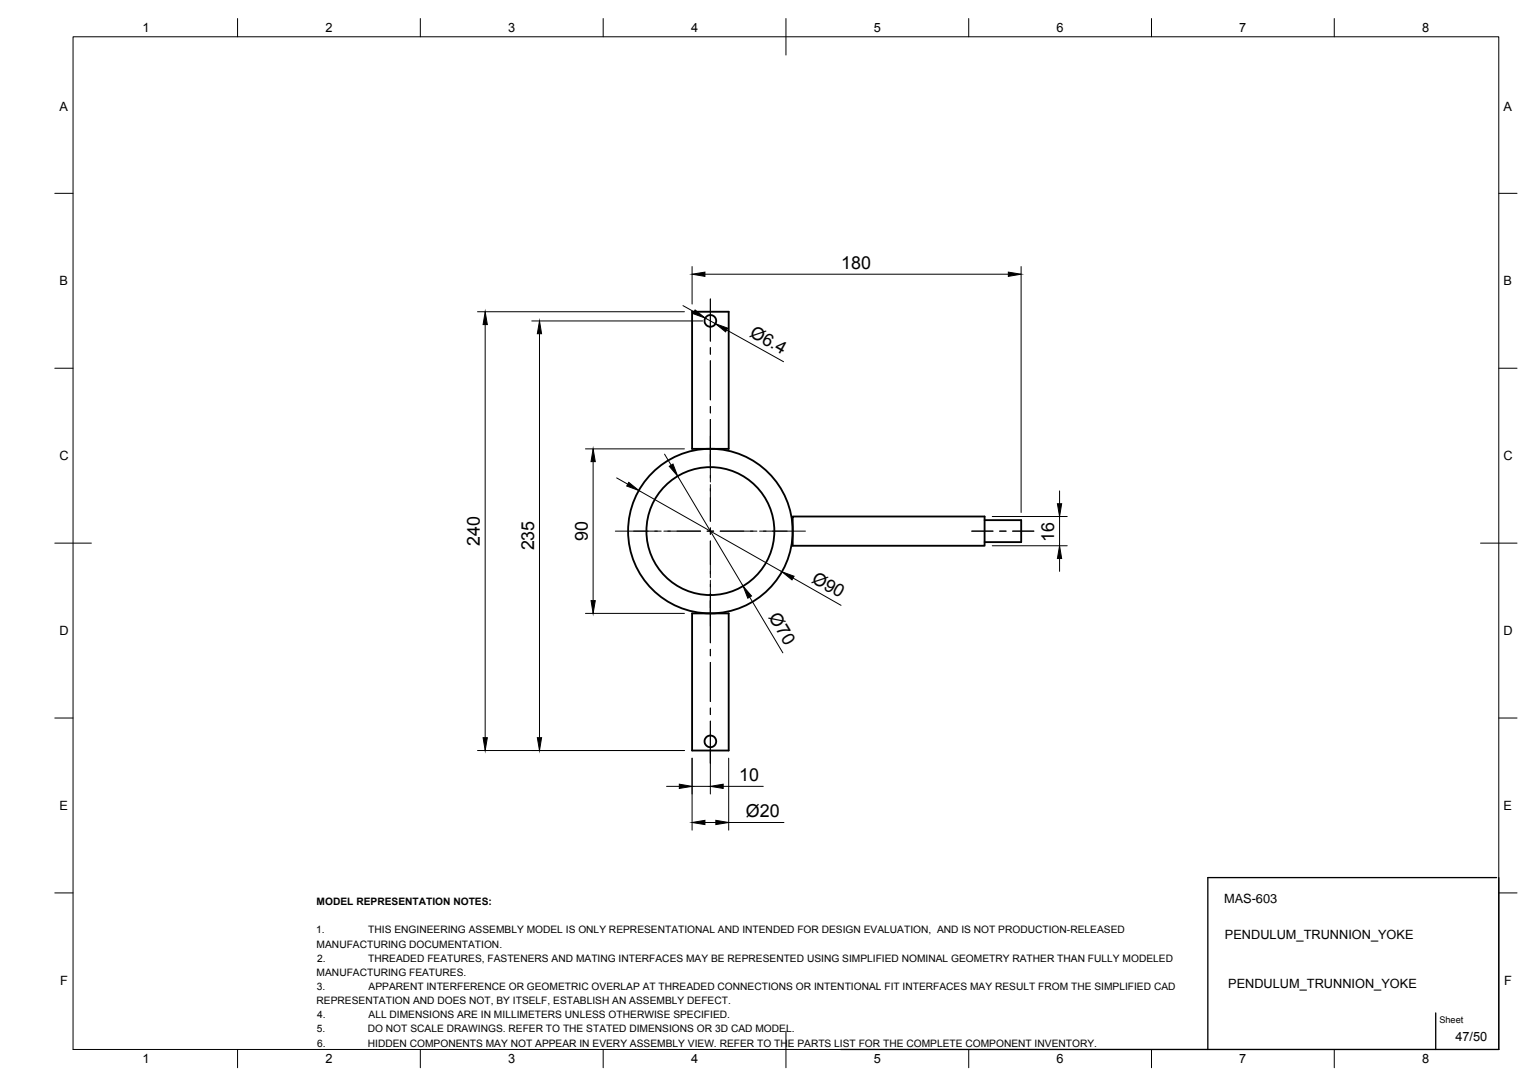
ISO-10303-21;
HEADER;
FILE_DESCRIPTION((''),'2;1');
FILE_NAME('PENDULUM_TRUNNION_YOKE.step','2026-10-01T22:06:14-07:00',(''),(''),'','','');
FILE_SCHEMA (('AUTOMOTIVE_DESIGN { 1 0 10303 214 3 1 1 }'));
ENDSEC;
DATA;
#10=MECHANICAL_DESIGN_GEOMETRIC_PRESENTATION_REPRESENTATION('',(#1022,#1023,#1024,#1025),#50440);
#38=B_SPLINE_CURVE_WITH_KNOTS('',3,(#49556,#49557,#49558,#49559,#49560,
#49561,#49562,#49563,#49564,#49565,#49566,#49567,#49568,#49569,#49570,#49571,
#49572,#49573,#49574),.UNSPECIFIED.,.F.,.F.,(4,2,2,2,3,2,2,2,4),(1.45762049263555,
1.57906514727215,1.70050980190876,1.82200189604475,1.94349399018073,2.06498608431671,
2.18647817845269,2.3079228330893,2.42936748772591),.UNSPECIFIED.) ;
#39=B_SPLINE_CURVE_WITH_KNOTS('',3,(#49577,#49578,#49579,#49580,#49581,
#49582,#49583,#49584,#49585,#49586,#49587,#49588,#49589,#49590,#49591,#49592,
#49593,#49594),.UNSPECIFIED.,.F.,.F.,(4,2,2,2,2,2,2,2,4),(0.485873497545182,
0.60731815218179,0.728762806818399,0.850254900954381,0.971746995090364,
1.09323908922635,1.21473118336233,1.33617583799894,1.45762049263555),
 .UNSPECIFIED.) ;
#40=B_SPLINE_CURVE_WITH_KNOTS('',3,(#49597,#49598,#49599,#49600,#49601,
#49602,#49603,#49604,#49605,#49606,#49607,#49608,#49609,#49610,#49611,#49612,
#49613,#49614),.UNSPECIFIED.,.F.,.F.,(4,2,2,2,2,2,2,2,4),(0.485873497545182,
0.607318152181791,0.728762806818399,0.850254900954382,0.971746995090364,
1.09323908922635,1.21473118336233,1.33617583799894,1.45762049263555),
 .UNSPECIFIED.) ;
#41=B_SPLINE_CURVE_WITH_KNOTS('',3,(#49615,#49616,#49617,#49618,#49619,
#49620,#49621,#49622,#49623,#49624,#49625,#49626,#49627,#49628,#49629,#49630,
#49631,#49632,#49633),.UNSPECIFIED.,.F.,.F.,(4,2,2,2,3,2,2,2,4),(1.45762049263555,
1.57906514727215,1.70050980190876,1.82200189604475,1.94349399018073,2.06498608431671,
2.18647817845269,2.3079228330893,2.42936748772591),.UNSPECIFIED.) ;
#42=B_SPLINE_CURVE_WITH_KNOTS('',3,(#49640,#49641,#49642,#49643,#49644,
#49645,#49646,#49647,#49648,#49649,#49650,#49651,#49652,#49653,#49654,#49655,
#49656,#49657),.UNSPECIFIED.,.F.,.F.,(4,2,2,2,2,2,2,2,4),(0.485873497545182,
0.607318152181791,0.728762806818399,0.850254900954382,0.971746995090364,
1.09323908922635,1.21473118336233,1.33617583799894,1.45762049263555),
 .UNSPECIFIED.) ;
#43=B_SPLINE_CURVE_WITH_KNOTS('',3,(#49658,#49659,#49660,#49661,#49662,
#49663,#49664,#49665,#49666,#49667,#49668,#49669,#49670,#49671,#49672,#49673,
#49674,#49675,#49676),.UNSPECIFIED.,.F.,.F.,(4,2,2,2,3,2,2,2,4),(1.45762049263555,
1.57906514727215,1.70050980190876,1.82200189604475,1.94349399018073,2.06498608431671,
2.18647817845269,2.3079228330893,2.42936748772591),.UNSPECIFIED.) ;
#44=B_SPLINE_CURVE_WITH_KNOTS('',3,(#49680,#49681,#49682,#49683,#49684,
#49685,#49686,#49687,#49688,#49689,#49690,#49691,#49692,#49693,#49694,#49695,
#49696,#49697,#49698),.UNSPECIFIED.,.F.,.F.,(4,2,2,2,3,2,2,2,4),(1.45762049263555,
1.57906514727215,1.70050980190876,1.82200189604475,1.94349399018073,2.06498608431671,
2.18647817845269,2.3079228330893,2.42936748772591),.UNSPECIFIED.) ;
#45=B_SPLINE_CURVE_WITH_KNOTS('',3,(#49699,#49700,#49701,#49702,#49703,
#49704,#49705,#49706,#49707,#49708,#49709,#49710,#49711,#49712,#49713,#49714,
#49715,#49716),.UNSPECIFIED.,.F.,.F.,(4,2,2,2,2,2,2,2,4),(0.485873497545182,
0.60731815218179,0.728762806818399,0.850254900954381,0.971746995090364,
1.09323908922635,1.21473118336233,1.33617583799894,1.45762049263555),
 .UNSPECIFIED.) ;
#925=SHAPE_REPRESENTATION_RELATIONSHIP('SRR','None',#50659,#970) ;
#970=ADVANCED_BREP_SHAPE_REPRESENTATION('',(#1075,#1076,#1077,#1078),#50428) ;
#1022=STYLED_ITEM('',(#50883),#1075) ;
#1023=STYLED_ITEM('',(#50883),#1076) ;
#1024=STYLED_ITEM('',(#50883),#1077) ;
#1025=STYLED_ITEM('',(#50883),#1078) ;
#1075=MANIFOLD_SOLID_BREP('PENDULUM_TRUNNION_YOKE',#28700) ;
#1076=MANIFOLD_SOLID_BREP('PENDULUM_TRUNNION_YOKE',#28701) ;
#1077=MANIFOLD_SOLID_BREP('PENDULUM_TRUNNION_YOKE',#28702) ;
#1078=MANIFOLD_SOLID_BREP('PENDULUM_TRUNNION_YOKE',#28703) ;
#1390=FACE_BOUND('',#5605,.T.) ;
#1391=FACE_BOUND('',#5612,.T.) ;
#1392=FACE_BOUND('',#5618,.T.) ;
#1393=FACE_BOUND('',#5622,.T.) ;
#1394=FACE_BOUND('',#5624,.T.) ;
#1395=FACE_BOUND('',#5626,.T.) ;
#2258=PLANE('',#32122) ;
#2259=PLANE('',#32123) ;
#2260=PLANE('',#32124) ;
#2261=PLANE('',#32125) ;
#2262=PLANE('',#32126) ;
#2263=PLANE('',#32127) ;
#2264=PLANE('',#32128) ;
#2265=PLANE('',#32129) ;
#2266=PLANE('',#32130) ;
#2267=PLANE('',#32132) ;
#2268=PLANE('',#32136) ;
#2269=PLANE('',#32139) ;
#2270=PLANE('',#32144) ;
#2271=PLANE('',#32145) ;
#2272=PLANE('',#32149) ;
#2273=PLANE('',#32152) ;
#3767=FACE_OUTER_BOUND('',#5599,.T.) ;
#3768=FACE_OUTER_BOUND('',#5600,.T.) ;
#3769=FACE_OUTER_BOUND('',#5601,.T.) ;
#3770=FACE_OUTER_BOUND('',#5602,.T.) ;
#3771=FACE_OUTER_BOUND('',#5603,.T.) ;
#3772=FACE_OUTER_BOUND('',#5604,.T.) ;
#3773=FACE_OUTER_BOUND('',#5606,.T.) ;
#3774=FACE_OUTER_BOUND('',#5607,.T.) ;
#3775=FACE_OUTER_BOUND('',#5608,.T.) ;
#3776=FACE_OUTER_BOUND('',#5609,.T.) ;
#3777=FACE_OUTER_BOUND('',#5610,.T.) ;
#3778=FACE_OUTER_BOUND('',#5611,.T.) ;
#3779=FACE_OUTER_BOUND('',#5613,.T.) ;
#3780=FACE_OUTER_BOUND('',#5614,.T.) ;
#3781=FACE_OUTER_BOUND('',#5615,.T.) ;
#3782=FACE_OUTER_BOUND('',#5616,.T.) ;
#3783=FACE_OUTER_BOUND('',#5617,.T.) ;
#3784=FACE_OUTER_BOUND('',#5619,.T.) ;
#3785=FACE_OUTER_BOUND('',#5620,.T.) ;
#3786=FACE_OUTER_BOUND('',#5621,.T.) ;
#3787=FACE_OUTER_BOUND('',#5623,.T.) ;
#3788=FACE_OUTER_BOUND('',#5625,.T.) ;
#3789=FACE_OUTER_BOUND('',#5627,.T.) ;
#3790=FACE_OUTER_BOUND('',#5628,.T.) ;
#5599=EDGE_LOOP('',(#26079,#26080,#26081,#26082)) ;
#5600=EDGE_LOOP('',(#26083)) ;
#5601=EDGE_LOOP('',(#26084,#26085,#26086,#26087)) ;
#5602=EDGE_LOOP('',(#26088,#26089,#26090,#26091,#26092)) ;
#5603=EDGE_LOOP('',(#26093,#26094,#26095,#26096,#26097)) ;
#5604=EDGE_LOOP('',(#26098,#26099,#26100,#26101)) ;
#5605=EDGE_LOOP('',(#26102)) ;
#5606=EDGE_LOOP('',(#26103,#26104,#26105,#26106)) ;
#5607=EDGE_LOOP('',(#26107,#26108,#26109,#26110)) ;
#5608=EDGE_LOOP('',(#26111,#26112,#26113,#26114)) ;
#5609=EDGE_LOOP('',(#26115)) ;
#5610=EDGE_LOOP('',(#26116,#26117)) ;
#5611=EDGE_LOOP('',(#26118,#26119,#26120,#26121,#26122,#26123,#26124,#26125,
#26126)) ;
#5612=EDGE_LOOP('',(#26127,#26128)) ;
#5613=EDGE_LOOP('',(#26129,#26130)) ;
#5614=EDGE_LOOP('',(#26131,#26132,#26133,#26134,#26135,#26136)) ;
#5615=EDGE_LOOP('',(#26137,#26138,#26139,#26140,#26141,#26142)) ;
#5616=EDGE_LOOP('',(#26143,#26144)) ;
#5617=EDGE_LOOP('',(#26145,#26146,#26147,#26148,#26149,#26150,#26151,#26152,
#26153)) ;
#5618=EDGE_LOOP('',(#26154,#26155)) ;
#5619=EDGE_LOOP('',(#26156)) ;
#5620=EDGE_LOOP('',(#26157,#26158)) ;
#5621=EDGE_LOOP('',(#26159,#26160,#26161,#26162,#26163,#26164,#26165,#26166)) ;
#5622=EDGE_LOOP('',(#26167,#26168)) ;
#5623=EDGE_LOOP('',(#26169,#26170)) ;
#5624=EDGE_LOOP('',(#26171)) ;
#5625=EDGE_LOOP('',(#26172,#26173)) ;
#5626=EDGE_LOOP('',(#26174)) ;
#5627=EDGE_LOOP('',(#26175,#26176,#26177,#26178,#26179,#26180,#26181,#26182)) ;
#5628=EDGE_LOOP('',(#26183,#26184,#26185,#26186)) ;
#8043=LINE('',#49509,#10515) ;
#8044=LINE('',#49515,#10516) ;
#8045=LINE('',#49517,#10517) ;
#8046=LINE('',#49519,#10518) ;
#8047=LINE('',#49520,#10519) ;
#8048=LINE('',#49524,#10520) ;
#8049=LINE('',#49525,#10521) ;
#8050=LINE('',#49527,#10522) ;
#8051=LINE('',#49528,#10523) ;
#8052=LINE('',#49532,#10524) ;
#8053=LINE('',#49534,#10525) ;
#8054=LINE('',#49535,#10526) ;
#8055=LINE('',#49536,#10527) ;
#8056=LINE('',#49538,#10528) ;
#8057=LINE('',#49539,#10529) ;
#8058=LINE('',#49542,#10530) ;
#8059=LINE('',#49550,#10531) ;
#8060=LINE('',#49554,#10532) ;
#8061=LINE('',#49575,#10533) ;
#8062=LINE('',#49636,#10534) ;
#8063=LINE('',#49678,#10535) ;
#8064=LINE('',#49720,#10536) ;
#8065=LINE('',#49724,#10537) ;
#8066=LINE('',#49726,#10538) ;
#8067=LINE('',#49733,#10539) ;
#8068=LINE('',#49735,#10540) ;
#8069=LINE('',#49737,#10541) ;
#8070=LINE('',#49741,#10542) ;
#8071=LINE('',#49743,#10543) ;
#8072=LINE('',#49745,#10544) ;
#8073=LINE('',#49749,#10545) ;
#8074=LINE('',#49760,#10546) ;
#10515=VECTOR('',#40510,0.6) ;
#10516=VECTOR('',#40517,1.) ;
#10517=VECTOR('',#40518,1.) ;
#10518=VECTOR('',#40519,1.) ;
#10519=VECTOR('',#40520,1.) ;
#10520=VECTOR('',#40523,1.) ;
#10521=VECTOR('',#40524,1.) ;
#10522=VECTOR('',#40525,1.) ;
#10523=VECTOR('',#40526,1.) ;
#10524=VECTOR('',#40529,1.) ;
#10525=VECTOR('',#40530,1.) ;
#10526=VECTOR('',#40531,1.) ;
#10527=VECTOR('',#40532,1.) ;
#10528=VECTOR('',#40535,1.) ;
#10529=VECTOR('',#40536,1.) ;
#10530=VECTOR('',#40541,1.) ;
#10531=VECTOR('',#40550,1.) ;
#10532=VECTOR('',#40555,1.) ;
#10533=VECTOR('',#40556,1.) ;
#10534=VECTOR('',#40563,0.32) ;
#10535=VECTOR('',#40566,0.32) ;
#10536=VECTOR('',#40569,1.) ;
#10537=VECTOR('',#40576,1.) ;
#10538=VECTOR('',#40577,1.) ;
#10539=VECTOR('',#40586,4.5) ;
#10540=VECTOR('',#40587,1.) ;
#10541=VECTOR('',#40588,4.5) ;
#10542=VECTOR('',#40591,4.5) ;
#10543=VECTOR('',#40592,1.) ;
#10544=VECTOR('',#40593,4.5) ;
#10545=VECTOR('',#40596,1.) ;
#10546=VECTOR('',#40613,3.5) ;
#11777=CIRCLE('',#32120,0.6) ;
#11778=CIRCLE('',#32121,0.6) ;
#11779=CIRCLE('',#32131,1.) ;
#11780=CIRCLE('',#32133,1.) ;
#11781=CIRCLE('',#32135,1.) ;
#11782=CIRCLE('',#32140,1.) ;
#11783=CIRCLE('',#32142,1.) ;
#11784=CIRCLE('',#32143,1.) ;
#11785=CIRCLE('',#32147,4.5) ;
#11786=CIRCLE('',#32148,4.5) ;
#11787=CIRCLE('',#32150,4.5) ;
#11788=CIRCLE('',#32151,3.5) ;
#11789=CIRCLE('',#32153,4.5) ;
#11790=CIRCLE('',#32154,3.5) ;
#14370=VERTEX_POINT('',#49506) ;
#14371=VERTEX_POINT('',#49508) ;
#14372=VERTEX_POINT('',#49513) ;
#14373=VERTEX_POINT('',#49514) ;
#14374=VERTEX_POINT('',#49516) ;
#14375=VERTEX_POINT('',#49518) ;
#14376=VERTEX_POINT('',#49522) ;
#14377=VERTEX_POINT('',#49523) ;
#14378=VERTEX_POINT('',#49526) ;
#14379=VERTEX_POINT('',#49530) ;
#14380=VERTEX_POINT('',#49531) ;
#14381=VERTEX_POINT('',#49533) ;
#14382=VERTEX_POINT('',#49545) ;
#14383=VERTEX_POINT('',#49548) ;
#14384=VERTEX_POINT('',#49549) ;
#14385=VERTEX_POINT('',#49553) ;
#14386=VERTEX_POINT('',#49555) ;
#14387=VERTEX_POINT('',#49595) ;
#14388=VERTEX_POINT('',#49596) ;
#14389=VERTEX_POINT('',#49638) ;
#14390=VERTEX_POINT('',#49639) ;
#14391=VERTEX_POINT('',#49677) ;
#14392=VERTEX_POINT('',#49679) ;
#14393=VERTEX_POINT('',#49718) ;
#14394=VERTEX_POINT('',#49719) ;
#14395=VERTEX_POINT('',#49725) ;
#14396=VERTEX_POINT('',#49731) ;
#14397=VERTEX_POINT('',#49732) ;
#14398=VERTEX_POINT('',#49734) ;
#14399=VERTEX_POINT('',#49736) ;
#14400=VERTEX_POINT('',#49738) ;
#14401=VERTEX_POINT('',#49740) ;
#14402=VERTEX_POINT('',#49742) ;
#14403=VERTEX_POINT('',#49744) ;
#14404=VERTEX_POINT('',#49747) ;
#14405=VERTEX_POINT('',#49748) ;
#14406=VERTEX_POINT('',#49752) ;
#14407=VERTEX_POINT('',#49756) ;
#18305=EDGE_CURVE('',#14370,#14370,#11777,.T.) ;
#18306=EDGE_CURVE('',#14370,#14371,#8043,.T.) ;
#18307=EDGE_CURVE('',#14371,#14371,#11778,.T.) ;
#18308=EDGE_CURVE('',#14372,#14373,#8044,.T.) ;
#18309=EDGE_CURVE('',#14374,#14372,#8045,.T.) ;
#18310=EDGE_CURVE('',#14375,#14374,#8046,.T.) ;
#18311=EDGE_CURVE('',#14373,#14375,#8047,.T.) ;
#18312=EDGE_CURVE('',#14376,#14377,#8048,.T.) ;
#18313=EDGE_CURVE('',#14377,#14373,#8049,.T.) ;
#18314=EDGE_CURVE('',#14375,#14378,#8050,.T.) ;
#18315=EDGE_CURVE('',#14378,#14376,#8051,.T.) ;
#18316=EDGE_CURVE('',#14379,#14380,#8052,.T.) ;
#18317=EDGE_CURVE('',#14380,#14381,#8053,.T.) ;
#18318=EDGE_CURVE('',#14381,#14374,#8054,.T.) ;
#18319=EDGE_CURVE('',#14372,#14379,#8055,.T.) ;
#18320=EDGE_CURVE('',#14378,#14381,#8056,.T.) ;
#18321=EDGE_CURVE('',#14376,#14380,#8057,.T.) ;
#18322=EDGE_CURVE('',#14377,#14379,#8058,.T.) ;
#18323=EDGE_CURVE('',#14382,#14382,#11779,.T.) ;
#18324=EDGE_CURVE('',#14383,#14384,#8059,.T.) ;
#18325=EDGE_CURVE('',#14384,#14383,#11780,.T.) ;
#18326=EDGE_CURVE('',#14382,#14385,#8060,.T.) ;
#18327=EDGE_CURVE('',#14385,#14386,#38,.T.) ;
#18328=EDGE_CURVE('',#14386,#14384,#8061,.T.) ;
#18329=EDGE_CURVE('',#14383,#14384,#11781,.T.) ;
#18330=EDGE_CURVE('',#14386,#14385,#39,.T.) ;
#18331=EDGE_CURVE('',#14387,#14388,#40,.T.) ;
#18332=EDGE_CURVE('',#14388,#14387,#41,.T.) ;
#18333=EDGE_CURVE('',#14388,#14386,#8062,.T.) ;
#18334=EDGE_CURVE('',#14389,#14390,#42,.T.) ;
#18335=EDGE_CURVE('',#14390,#14389,#43,.T.) ;
#18336=EDGE_CURVE('',#14390,#14391,#8063,.T.) ;
#18337=EDGE_CURVE('',#14392,#14391,#44,.T.) ;
#18338=EDGE_CURVE('',#14391,#14392,#45,.T.) ;
#18339=EDGE_CURVE('',#14393,#14394,#8064,.T.) ;
#18340=EDGE_CURVE('',#14393,#14394,#11782,.T.) ;
#18341=EDGE_CURVE('',#14394,#14393,#11783,.T.) ;
#18342=EDGE_CURVE('',#14394,#14392,#8065,.T.) ;
#18343=EDGE_CURVE('',#14391,#14395,#8066,.T.) ;
#18344=EDGE_CURVE('',#14395,#14395,#11784,.T.) ;
#18345=EDGE_CURVE('',#14396,#14397,#8067,.T.) ;
#18346=EDGE_CURVE('',#14398,#14396,#8068,.T.) ;
#18347=EDGE_CURVE('',#14399,#14398,#8069,.T.) ;
#18348=EDGE_CURVE('',#14400,#14399,#11785,.T.) ;
#18349=EDGE_CURVE('',#14401,#14400,#8070,.T.) ;
#18350=EDGE_CURVE('',#14401,#14402,#8071,.T.) ;
#18351=EDGE_CURVE('',#14403,#14402,#8072,.T.) ;
#18352=EDGE_CURVE('',#14397,#14403,#11786,.T.) ;
#18353=EDGE_CURVE('',#14404,#14405,#8073,.T.) ;
#18354=EDGE_CURVE('',#14403,#14397,#11787,.T.) ;
#18355=EDGE_CURVE('',#14406,#14406,#11788,.T.) ;
#18356=EDGE_CURVE('',#14399,#14400,#11789,.T.) ;
#18357=EDGE_CURVE('',#14407,#14407,#11790,.T.) ;
#18358=EDGE_CURVE('',#14407,#14406,#8074,.T.) ;
#26079=ORIENTED_EDGE('',*,*,#18305,.F.) ;
#26080=ORIENTED_EDGE('',*,*,#18306,.T.) ;
#26081=ORIENTED_EDGE('',*,*,#18307,.F.) ;
#26082=ORIENTED_EDGE('',*,*,#18306,.F.) ;
#26083=ORIENTED_EDGE('',*,*,#18307,.T.) ;
#26084=ORIENTED_EDGE('',*,*,#18308,.F.) ;
#26085=ORIENTED_EDGE('',*,*,#18309,.F.) ;
#26086=ORIENTED_EDGE('',*,*,#18310,.F.) ;
#26087=ORIENTED_EDGE('',*,*,#18311,.F.) ;
#26088=ORIENTED_EDGE('',*,*,#18312,.T.) ;
#26089=ORIENTED_EDGE('',*,*,#18313,.T.) ;
#26090=ORIENTED_EDGE('',*,*,#18311,.T.) ;
#26091=ORIENTED_EDGE('',*,*,#18314,.T.) ;
#26092=ORIENTED_EDGE('',*,*,#18315,.T.) ;
#26093=ORIENTED_EDGE('',*,*,#18316,.T.) ;
#26094=ORIENTED_EDGE('',*,*,#18317,.T.) ;
#26095=ORIENTED_EDGE('',*,*,#18318,.T.) ;
#26096=ORIENTED_EDGE('',*,*,#18309,.T.) ;
#26097=ORIENTED_EDGE('',*,*,#18319,.T.) ;
#26098=ORIENTED_EDGE('',*,*,#18320,.T.) ;
#26099=ORIENTED_EDGE('',*,*,#18317,.F.) ;
#26100=ORIENTED_EDGE('',*,*,#18321,.F.) ;
#26101=ORIENTED_EDGE('',*,*,#18315,.F.) ;
#26102=ORIENTED_EDGE('',*,*,#18305,.T.) ;
#26103=ORIENTED_EDGE('',*,*,#18310,.T.) ;
#26104=ORIENTED_EDGE('',*,*,#18318,.F.) ;
#26105=ORIENTED_EDGE('',*,*,#18320,.F.) ;
#26106=ORIENTED_EDGE('',*,*,#18314,.F.) ;
#26107=ORIENTED_EDGE('',*,*,#18308,.T.) ;
#26108=ORIENTED_EDGE('',*,*,#18313,.F.) ;
#26109=ORIENTED_EDGE('',*,*,#18322,.T.) ;
#26110=ORIENTED_EDGE('',*,*,#18319,.F.) ;
#26111=ORIENTED_EDGE('',*,*,#18321,.T.) ;
#26112=ORIENTED_EDGE('',*,*,#18316,.F.) ;
#26113=ORIENTED_EDGE('',*,*,#18322,.F.) ;
#26114=ORIENTED_EDGE('',*,*,#18312,.F.) ;
#26115=ORIENTED_EDGE('',*,*,#18323,.T.) ;
#26116=ORIENTED_EDGE('',*,*,#18324,.T.) ;
#26117=ORIENTED_EDGE('',*,*,#18325,.T.) ;
#26118=ORIENTED_EDGE('',*,*,#18323,.F.) ;
#26119=ORIENTED_EDGE('',*,*,#18326,.T.) ;
#26120=ORIENTED_EDGE('',*,*,#18327,.T.) ;
#26121=ORIENTED_EDGE('',*,*,#18328,.T.) ;
#26122=ORIENTED_EDGE('',*,*,#18329,.F.) ;
#26123=ORIENTED_EDGE('',*,*,#18325,.F.) ;
#26124=ORIENTED_EDGE('',*,*,#18328,.F.) ;
#26125=ORIENTED_EDGE('',*,*,#18330,.T.) ;
#26126=ORIENTED_EDGE('',*,*,#18326,.F.) ;
#26127=ORIENTED_EDGE('',*,*,#18331,.T.) ;
#26128=ORIENTED_EDGE('',*,*,#18332,.T.) ;
#26129=ORIENTED_EDGE('',*,*,#18324,.F.) ;
#26130=ORIENTED_EDGE('',*,*,#18329,.T.) ;
#26131=ORIENTED_EDGE('',*,*,#18331,.F.) ;
#26132=ORIENTED_EDGE('',*,*,#18332,.F.) ;
#26133=ORIENTED_EDGE('',*,*,#18333,.T.) ;
#26134=ORIENTED_EDGE('',*,*,#18327,.F.) ;
#26135=ORIENTED_EDGE('',*,*,#18330,.F.) ;
#26136=ORIENTED_EDGE('',*,*,#18333,.F.) ;
#26137=ORIENTED_EDGE('',*,*,#18334,.F.) ;
#26138=ORIENTED_EDGE('',*,*,#18335,.F.) ;
#26139=ORIENTED_EDGE('',*,*,#18336,.T.) ;
#26140=ORIENTED_EDGE('',*,*,#18337,.F.) ;
#26141=ORIENTED_EDGE('',*,*,#18338,.F.) ;
#26142=ORIENTED_EDGE('',*,*,#18336,.F.) ;
#26143=ORIENTED_EDGE('',*,*,#18339,.F.) ;
#26144=ORIENTED_EDGE('',*,*,#18340,.T.) ;
#26145=ORIENTED_EDGE('',*,*,#18340,.F.) ;
#26146=ORIENTED_EDGE('',*,*,#18341,.F.) ;
#26147=ORIENTED_EDGE('',*,*,#18342,.T.) ;
#26148=ORIENTED_EDGE('',*,*,#18337,.T.) ;
#26149=ORIENTED_EDGE('',*,*,#18343,.T.) ;
#26150=ORIENTED_EDGE('',*,*,#18344,.F.) ;
#26151=ORIENTED_EDGE('',*,*,#18343,.F.) ;
#26152=ORIENTED_EDGE('',*,*,#18338,.T.) ;
#26153=ORIENTED_EDGE('',*,*,#18342,.F.) ;
#26154=ORIENTED_EDGE('',*,*,#18334,.T.) ;
#26155=ORIENTED_EDGE('',*,*,#18335,.T.) ;
#26156=ORIENTED_EDGE('',*,*,#18344,.T.) ;
#26157=ORIENTED_EDGE('',*,*,#18339,.T.) ;
#26158=ORIENTED_EDGE('',*,*,#18341,.T.) ;
#26159=ORIENTED_EDGE('',*,*,#18345,.F.) ;
#26160=ORIENTED_EDGE('',*,*,#18346,.F.) ;
#26161=ORIENTED_EDGE('',*,*,#18347,.F.) ;
#26162=ORIENTED_EDGE('',*,*,#18348,.F.) ;
#26163=ORIENTED_EDGE('',*,*,#18349,.F.) ;
#26164=ORIENTED_EDGE('',*,*,#18350,.T.) ;
#26165=ORIENTED_EDGE('',*,*,#18351,.F.) ;
#26166=ORIENTED_EDGE('',*,*,#18352,.F.) ;
#26167=ORIENTED_EDGE('',*,*,#18353,.T.) ;
#26168=ORIENTED_EDGE('',*,*,#18353,.F.) ;
#26169=ORIENTED_EDGE('',*,*,#18354,.T.) ;
#26170=ORIENTED_EDGE('',*,*,#18352,.T.) ;
#26171=ORIENTED_EDGE('',*,*,#18355,.T.) ;
#26172=ORIENTED_EDGE('',*,*,#18348,.T.) ;
#26173=ORIENTED_EDGE('',*,*,#18356,.T.) ;
#26174=ORIENTED_EDGE('',*,*,#18357,.T.) ;
#26175=ORIENTED_EDGE('',*,*,#18345,.T.) ;
#26176=ORIENTED_EDGE('',*,*,#18354,.F.) ;
#26177=ORIENTED_EDGE('',*,*,#18351,.T.) ;
#26178=ORIENTED_EDGE('',*,*,#18350,.F.) ;
#26179=ORIENTED_EDGE('',*,*,#18349,.T.) ;
#26180=ORIENTED_EDGE('',*,*,#18356,.F.) ;
#26181=ORIENTED_EDGE('',*,*,#18347,.T.) ;
#26182=ORIENTED_EDGE('',*,*,#18346,.T.) ;
#26183=ORIENTED_EDGE('',*,*,#18357,.F.) ;
#26184=ORIENTED_EDGE('',*,*,#18358,.T.) ;
#26185=ORIENTED_EDGE('',*,*,#18355,.F.) ;
#26186=ORIENTED_EDGE('',*,*,#18358,.F.) ;
#27041=CYLINDRICAL_SURFACE('',#32119,0.6) ;
#27042=CYLINDRICAL_SURFACE('',#32134,1.) ;
#27043=CYLINDRICAL_SURFACE('',#32137,0.32) ;
#27044=CYLINDRICAL_SURFACE('',#32138,0.32) ;
#27045=CYLINDRICAL_SURFACE('',#32141,1.) ;
#27046=CYLINDRICAL_SURFACE('',#32146,4.5) ;
#27047=CYLINDRICAL_SURFACE('',#32155,4.5) ;
#27048=CYLINDRICAL_SURFACE('',#32156,3.5) ;
#28502=ADVANCED_FACE('',(#3767),#27041,.T.) ;
#28503=ADVANCED_FACE('',(#3768),#2258,.T.) ;
#28504=ADVANCED_FACE('',(#3769),#2259,.F.) ;
#28505=ADVANCED_FACE('',(#3770),#2260,.T.) ;
#28506=ADVANCED_FACE('',(#3771),#2261,.F.) ;
#28507=ADVANCED_FACE('',(#3772,#1390),#2262,.F.) ;
#28508=ADVANCED_FACE('',(#3773),#2263,.F.) ;
#28509=ADVANCED_FACE('',(#3774),#2264,.F.) ;
#28510=ADVANCED_FACE('',(#3775),#2265,.F.) ;
#28511=ADVANCED_FACE('',(#3776),#2266,.T.) ;
#28512=ADVANCED_FACE('',(#3777),#2267,.T.) ;
#28513=ADVANCED_FACE('',(#3778,#1391),#27042,.T.) ;
#28514=ADVANCED_FACE('',(#3779),#2268,.T.) ;
#28515=ADVANCED_FACE('',(#3780),#27043,.F.) ;
#28516=ADVANCED_FACE('',(#3781),#27044,.F.) ;
#28517=ADVANCED_FACE('',(#3782),#2269,.T.) ;
#28518=ADVANCED_FACE('',(#3783,#1392),#27045,.T.) ;
#28519=ADVANCED_FACE('',(#3784),#2270,.T.) ;
#28520=ADVANCED_FACE('',(#3785),#2271,.T.) ;
#28521=ADVANCED_FACE('',(#3786,#1393),#27046,.T.) ;
#28522=ADVANCED_FACE('',(#3787,#1394),#2272,.T.) ;
#28523=ADVANCED_FACE('',(#3788,#1395),#2273,.T.) ;
#28524=ADVANCED_FACE('',(#3789),#27047,.T.) ;
#28525=ADVANCED_FACE('',(#3790),#27048,.F.) ;
#28700=CLOSED_SHELL('',(#28502,#28503,#28504,#28505,#28506,#28507,#28508,
#28509,#28510)) ;
#28701=CLOSED_SHELL('',(#28511,#28512,#28513,#28514,#28515)) ;
#28702=CLOSED_SHELL('',(#28516,#28517,#28518,#28519,#28520)) ;
#28703=CLOSED_SHELL('',(#28521,#28522,#28523,#28524,#28525)) ;
#32118=AXIS2_PLACEMENT_3D('',#49504,#40504,#40505) ;
#32119=AXIS2_PLACEMENT_3D('',#49505,#40506,#40507) ;
#32120=AXIS2_PLACEMENT_3D('',#49507,#40508,#40509) ;
#32121=AXIS2_PLACEMENT_3D('',#49510,#40511,#40512) ;
#32122=AXIS2_PLACEMENT_3D('',#49511,#40513,#40514) ;
#32123=AXIS2_PLACEMENT_3D('',#49512,#40515,#40516) ;
#32124=AXIS2_PLACEMENT_3D('',#49521,#40521,#40522) ;
#32125=AXIS2_PLACEMENT_3D('',#49529,#40527,#40528) ;
#32126=AXIS2_PLACEMENT_3D('',#49537,#40533,#40534) ;
#32127=AXIS2_PLACEMENT_3D('',#49540,#40537,#40538) ;
#32128=AXIS2_PLACEMENT_3D('',#49541,#40539,#40540) ;
#32129=AXIS2_PLACEMENT_3D('',#49543,#40542,#40543) ;
#32130=AXIS2_PLACEMENT_3D('',#49544,#40544,#40545) ;
#32131=AXIS2_PLACEMENT_3D('',#49546,#40546,#40547) ;
#32132=AXIS2_PLACEMENT_3D('',#49547,#40548,#40549) ;
#32133=AXIS2_PLACEMENT_3D('',#49551,#40551,#40552) ;
#32134=AXIS2_PLACEMENT_3D('',#49552,#40553,#40554) ;
#32135=AXIS2_PLACEMENT_3D('',#49576,#40557,#40558) ;
#32136=AXIS2_PLACEMENT_3D('',#49634,#40559,#40560) ;
#32137=AXIS2_PLACEMENT_3D('',#49635,#40561,#40562) ;
#32138=AXIS2_PLACEMENT_3D('',#49637,#40564,#40565) ;
#32139=AXIS2_PLACEMENT_3D('',#49717,#40567,#40568) ;
#32140=AXIS2_PLACEMENT_3D('',#49721,#40570,#40571) ;
#32141=AXIS2_PLACEMENT_3D('',#49722,#40572,#40573) ;
#32142=AXIS2_PLACEMENT_3D('',#49723,#40574,#40575) ;
#32143=AXIS2_PLACEMENT_3D('',#49727,#40578,#40579) ;
#32144=AXIS2_PLACEMENT_3D('',#49728,#40580,#40581) ;
#32145=AXIS2_PLACEMENT_3D('',#49729,#40582,#40583) ;
#32146=AXIS2_PLACEMENT_3D('',#49730,#40584,#40585) ;
#32147=AXIS2_PLACEMENT_3D('',#49739,#40589,#40590) ;
#32148=AXIS2_PLACEMENT_3D('',#49746,#40594,#40595) ;
#32149=AXIS2_PLACEMENT_3D('',#49750,#40597,#40598) ;
#32150=AXIS2_PLACEMENT_3D('',#49751,#40599,#40600) ;
#32151=AXIS2_PLACEMENT_3D('',#49753,#40601,#40602) ;
#32152=AXIS2_PLACEMENT_3D('',#49754,#40603,#40604) ;
#32153=AXIS2_PLACEMENT_3D('',#49755,#40605,#40606) ;
#32154=AXIS2_PLACEMENT_3D('',#49757,#40607,#40608) ;
#32155=AXIS2_PLACEMENT_3D('',#49758,#40609,#40610) ;
#32156=AXIS2_PLACEMENT_3D('',#49759,#40611,#40612) ;
#40504=DIRECTION('axis',(0.,0.,1.)) ;
#40505=DIRECTION('refdir',(1.,0.,0.)) ;
#40506=DIRECTION('center_axis',(0.,1.,0.)) ;
#40507=DIRECTION('ref_axis',(1.,0.,0.)) ;
#40508=DIRECTION('center_axis',(0.,1.,0.)) ;
#40509=DIRECTION('ref_axis',(1.,0.,0.)) ;
#40510=DIRECTION('',(0.,-1.,0.)) ;
#40511=DIRECTION('center_axis',(0.,-1.,0.)) ;
#40512=DIRECTION('ref_axis',(1.,0.,0.)) ;
#40513=DIRECTION('center_axis',(0.,-1.,0.)) ;
#40514=DIRECTION('ref_axis',(-1.,0.,0.)) ;
#40515=DIRECTION('center_axis',(0.,-1.,0.)) ;
#40516=DIRECTION('ref_axis',(0.,0.,-1.)) ;
#40517=DIRECTION('',(0.,0.,1.)) ;
#40518=DIRECTION('',(1.,0.,0.)) ;
#40519=DIRECTION('',(0.,0.,-1.)) ;
#40520=DIRECTION('',(-1.,0.,0.)) ;
#40521=DIRECTION('center_axis',(0.,0.,1.)) ;
#40522=DIRECTION('ref_axis',(1.,0.,0.)) ;
#40523=DIRECTION('',(0.,1.,0.)) ;
#40524=DIRECTION('',(-1.,0.,0.)) ;
#40525=DIRECTION('',(0.,-1.,0.)) ;
#40526=DIRECTION('',(1.,0.,0.)) ;
#40527=DIRECTION('center_axis',(0.,0.,1.)) ;
#40528=DIRECTION('ref_axis',(1.,0.,0.)) ;
#40529=DIRECTION('',(0.,-1.,0.)) ;
#40530=DIRECTION('',(-1.,0.,0.)) ;
#40531=DIRECTION('',(0.,1.,0.)) ;
#40532=DIRECTION('',(1.,0.,0.)) ;
#40533=DIRECTION('center_axis',(0.,1.,0.)) ;
#40534=DIRECTION('ref_axis',(0.,0.,1.)) ;
#40535=DIRECTION('',(0.,0.,-1.)) ;
#40536=DIRECTION('',(0.,0.,-1.)) ;
#40537=DIRECTION('center_axis',(1.,0.,0.)) ;
#40538=DIRECTION('ref_axis',(0.,0.,-1.)) ;
#40539=DIRECTION('center_axis',(0.,-1.,0.)) ;
#40540=DIRECTION('ref_axis',(0.,0.,-1.)) ;
#40541=DIRECTION('',(0.,0.,-1.)) ;
#40542=DIRECTION('center_axis',(-1.,0.,0.)) ;
#40543=DIRECTION('ref_axis',(0.,0.,1.)) ;
#40544=DIRECTION('center_axis',(1.,0.,0.)) ;
#40545=DIRECTION('ref_axis',(0.,0.,-1.)) ;
#40546=DIRECTION('center_axis',(1.,0.,0.)) ;
#40547=DIRECTION('ref_axis',(0.,0.,-1.)) ;
#40548=DIRECTION('center_axis',(-1.,0.,0.)) ;
#40549=DIRECTION('ref_axis',(0.,0.,1.)) ;
#40550=DIRECTION('',(0.,0.,1.)) ;
#40551=DIRECTION('center_axis',(-1.,0.,0.)) ;
#40552=DIRECTION('ref_axis',(0.,0.,-1.)) ;
#40553=DIRECTION('center_axis',(1.,0.,0.)) ;
#40554=DIRECTION('ref_axis',(0.,0.,-1.)) ;
#40555=DIRECTION('',(-1.,0.,0.)) ;
#40556=DIRECTION('',(-1.,0.,0.)) ;
#40557=DIRECTION('center_axis',(-1.,0.,0.)) ;
#40558=DIRECTION('ref_axis',(0.,0.,-1.)) ;
#40559=DIRECTION('center_axis',(-1.,0.,0.)) ;
#40560=DIRECTION('ref_axis',(0.,0.,1.)) ;
#40561=DIRECTION('center_axis',(0.,0.,1.)) ;
#40562=DIRECTION('ref_axis',(1.,0.,0.)) ;
#40563=DIRECTION('',(0.,0.,1.)) ;
#40564=DIRECTION('center_axis',(0.,0.,1.)) ;
#40565=DIRECTION('ref_axis',(1.,0.,0.)) ;
#40566=DIRECTION('',(0.,0.,1.)) ;
#40567=DIRECTION('center_axis',(1.,0.,0.)) ;
#40568=DIRECTION('ref_axis',(0.,0.,-1.)) ;
#40569=DIRECTION('',(0.,0.,1.)) ;
#40570=DIRECTION('center_axis',(1.,0.,0.)) ;
#40571=DIRECTION('ref_axis',(0.,0.,-1.)) ;
#40572=DIRECTION('center_axis',(1.,0.,0.)) ;
#40573=DIRECTION('ref_axis',(0.,0.,-1.)) ;
#40574=DIRECTION('center_axis',(1.,0.,0.)) ;
#40575=DIRECTION('ref_axis',(0.,0.,-1.)) ;
#40576=DIRECTION('',(-1.,0.,0.)) ;
#40577=DIRECTION('',(-1.,0.,0.)) ;
#40578=DIRECTION('center_axis',(-1.,0.,0.)) ;
#40579=DIRECTION('ref_axis',(0.,0.,-1.)) ;
#40580=DIRECTION('center_axis',(-1.,0.,0.)) ;
#40581=DIRECTION('ref_axis',(0.,0.,1.)) ;
#40582=DIRECTION('center_axis',(1.,0.,0.)) ;
#40583=DIRECTION('ref_axis',(0.,0.,-1.)) ;
#40584=DIRECTION('center_axis',(0.,0.,1.)) ;
#40585=DIRECTION('ref_axis',(6.12323399573677E-17,1.,0.)) ;
#40586=DIRECTION('',(0.,0.,1.)) ;
#40587=DIRECTION('',(0.,0.,1.)) ;
#40588=DIRECTION('',(0.,0.,1.)) ;
#40589=DIRECTION('center_axis',(0.,0.,-1.)) ;
#40590=DIRECTION('ref_axis',(1.,0.,0.)) ;
#40591=DIRECTION('',(0.,0.,-1.)) ;
#40592=DIRECTION('',(0.,0.,1.)) ;
#40593=DIRECTION('',(0.,0.,-1.)) ;
#40594=DIRECTION('center_axis',(0.,0.,1.)) ;
#40595=DIRECTION('ref_axis',(1.,0.,0.)) ;
#40596=DIRECTION('',(0.,0.,1.)) ;
#40597=DIRECTION('center_axis',(0.,0.,1.)) ;
#40598=DIRECTION('ref_axis',(1.,0.,0.)) ;
#40599=DIRECTION('center_axis',(0.,0.,1.)) ;
#40600=DIRECTION('ref_axis',(1.,0.,0.)) ;
#40601=DIRECTION('center_axis',(0.,0.,-1.)) ;
#40602=DIRECTION('ref_axis',(1.,0.,0.)) ;
#40603=DIRECTION('center_axis',(0.,0.,-1.)) ;
#40604=DIRECTION('ref_axis',(-1.,0.,0.)) ;
#40605=DIRECTION('center_axis',(0.,0.,-1.)) ;
#40606=DIRECTION('ref_axis',(1.,0.,0.)) ;
#40607=DIRECTION('center_axis',(0.,0.,1.)) ;
#40608=DIRECTION('ref_axis',(1.,0.,0.)) ;
#40609=DIRECTION('center_axis',(0.,0.,1.)) ;
#40610=DIRECTION('ref_axis',(6.12323399573677E-17,1.,0.)) ;
#40611=DIRECTION('center_axis',(0.,0.,1.)) ;
#40612=DIRECTION('ref_axis',(1.,0.,0.)) ;
#40613=DIRECTION('',(0.,0.,1.)) ;
#49504=CARTESIAN_POINT('',(0.,0.,0.)) ;
#49505=CARTESIAN_POINT('Origin',(0.,-16.,24.)) ;
#49506=CARTESIAN_POINT('',(-0.6,-15.,24.)) ;
#49507=CARTESIAN_POINT('Origin',(0.,-15.,24.)) ;
#49508=CARTESIAN_POINT('',(-0.6,-17.,24.)) ;
#49509=CARTESIAN_POINT('',(-0.6,-16.,24.)) ;
#49510=CARTESIAN_POINT('Origin',(0.,-17.,24.)) ;
#49511=CARTESIAN_POINT('Origin',(0.,-17.,24.)) ;
#49512=CARTESIAN_POINT('Origin',(0.,-4.5,24.)) ;
#49513=CARTESIAN_POINT('',(0.,-4.5,23.2)) ;
#49514=CARTESIAN_POINT('',(0.,-4.5,24.8)) ;
#49515=CARTESIAN_POINT('',(0.,-4.5,24.)) ;
#49516=CARTESIAN_POINT('',(-0.8,-4.5,23.2)) ;
#49517=CARTESIAN_POINT('',(0.,-4.5,23.2)) ;
#49518=CARTESIAN_POINT('',(-0.8,-4.5,24.8)) ;
#49519=CARTESIAN_POINT('',(-0.8,-4.5,24.)) ;
#49520=CARTESIAN_POINT('',(0.,-4.5,24.8)) ;
#49521=CARTESIAN_POINT('Origin',(0.,-9.75,24.8)) ;
#49522=CARTESIAN_POINT('',(0.8,-15.,24.8)) ;
#49523=CARTESIAN_POINT('',(0.8,-4.5,24.8)) ;
#49524=CARTESIAN_POINT('',(0.8,-9.75,24.8)) ;
#49525=CARTESIAN_POINT('',(0.,-4.5,24.8)) ;
#49526=CARTESIAN_POINT('',(-0.8,-15.,24.8)) ;
#49527=CARTESIAN_POINT('',(-0.8,-9.75,24.8)) ;
#49528=CARTESIAN_POINT('',(0.,-15.,24.8)) ;
#49529=CARTESIAN_POINT('Origin',(0.,-9.75,23.2)) ;
#49530=CARTESIAN_POINT('',(0.8,-4.5,23.2)) ;
#49531=CARTESIAN_POINT('',(0.8,-15.,23.2)) ;
#49532=CARTESIAN_POINT('',(0.8,-9.75,23.2)) ;
#49533=CARTESIAN_POINT('',(-0.8,-15.,23.2)) ;
#49534=CARTESIAN_POINT('',(0.,-15.,23.2)) ;
#49535=CARTESIAN_POINT('',(-0.8,-9.75,23.2)) ;
#49536=CARTESIAN_POINT('',(0.,-4.5,23.2)) ;
#49537=CARTESIAN_POINT('Origin',(0.,-15.,24.)) ;
#49538=CARTESIAN_POINT('',(-0.8,-15.,24.)) ;
#49539=CARTESIAN_POINT('',(0.8,-15.,24.)) ;
#49540=CARTESIAN_POINT('Origin',(-0.8,-9.75,24.)) ;
#49541=CARTESIAN_POINT('Origin',(0.,-4.5,24.)) ;
#49542=CARTESIAN_POINT('',(0.8,-4.5,24.)) ;
#49543=CARTESIAN_POINT('Origin',(0.8,-9.75,24.)) ;
#49544=CARTESIAN_POINT('Origin',(12.,0.,24.)) ;
#49545=CARTESIAN_POINT('',(12.,-1.22464679914735E-16,25.)) ;
#49546=CARTESIAN_POINT('Origin',(12.,0.,24.)) ;
#49547=CARTESIAN_POINT('Origin',(4.5,0.,24.)) ;
#49548=CARTESIAN_POINT('',(4.5,0.,23.)) ;
#49549=CARTESIAN_POINT('',(4.5,0.,25.)) ;
#49550=CARTESIAN_POINT('',(4.5,0.,24.)) ;
#49551=CARTESIAN_POINT('Origin',(4.5,0.,24.)) ;
#49552=CARTESIAN_POINT('Origin',(8.25,0.,24.)) ;
#49553=CARTESIAN_POINT('',(11.82,0.,25.)) ;
#49554=CARTESIAN_POINT('',(8.25,-1.22464679914735E-16,25.)) ;
#49555=CARTESIAN_POINT('',(11.18,0.,25.)) ;
#49556=CARTESIAN_POINT('Ctrl Pts',(11.82,0.,25.)) ;
#49557=CARTESIAN_POINT('Ctrl Pts',(11.82,-0.0404815515455362,25.)) ;
#49558=CARTESIAN_POINT('Ctrl Pts',(11.8118517942692,-0.0834711465257763,
24.9972999591064)) ;
#49559=CARTESIAN_POINT('Ctrl Pts',(11.7791044225004,-0.162233452253763,
24.9875499722835)) ;
#49560=CARTESIAN_POINT('Ctrl Pts',(11.7545204234507,-0.198027916508675,
24.9806252339521)) ;
#49561=CARTESIAN_POINT('Ctrl Pts',(11.6980168827738,-0.254531457185612,
24.9674995088223)) ;
#49562=CARTESIAN_POINT('Ctrl Pts',(11.6622268501742,-0.279106940985719,
24.9604129001751)) ;
#49563=CARTESIAN_POINT('Ctrl Pts',(11.583480842843,-0.311847989268857,24.9502865189927)) ;
#49564=CARTESIAN_POINT('Ctrl Pts',(11.540497364712,-0.32,24.9474175425862)) ;
#49565=CARTESIAN_POINT('Ctrl Pts',(11.5,-0.32,24.9474175425862)) ;
#49566=CARTESIAN_POINT('Ctrl Pts',(11.459502635288,-0.32,24.9474175425862)) ;
#49567=CARTESIAN_POINT('Ctrl Pts',(11.416519157157,-0.311847989268857,24.9502865189927)) ;
#49568=CARTESIAN_POINT('Ctrl Pts',(11.3377731498258,-0.279106940985719,
24.9604129001751)) ;
#49569=CARTESIAN_POINT('Ctrl Pts',(11.3019831172262,-0.254531457185612,
24.9674995088223)) ;
#49570=CARTESIAN_POINT('Ctrl Pts',(11.2454795765493,-0.198027916508675,
24.9806252339521)) ;
#49571=CARTESIAN_POINT('Ctrl Pts',(11.2208955774996,-0.162233452253763,
24.9875499722835)) ;
#49572=CARTESIAN_POINT('Ctrl Pts',(11.1881482057308,-0.0834711465257753,
24.9972999591064)) ;
#49573=CARTESIAN_POINT('Ctrl Pts',(11.18,-0.0404815515455361,25.)) ;
#49574=CARTESIAN_POINT('Ctrl Pts',(11.18,8.32667268468867E-17,25.)) ;
#49575=CARTESIAN_POINT('',(8.25,-1.22464679914735E-16,25.)) ;
#49576=CARTESIAN_POINT('Origin',(4.5,0.,24.)) ;
#49577=CARTESIAN_POINT('Ctrl Pts',(11.18,7.63278329429795E-17,25.)) ;
#49578=CARTESIAN_POINT('Ctrl Pts',(11.18,0.0404815515455362,25.)) ;
#49579=CARTESIAN_POINT('Ctrl Pts',(11.1881482057308,0.0834711465257764,
24.9972999591064)) ;
#49580=CARTESIAN_POINT('Ctrl Pts',(11.2208955774996,0.162233452253763,24.9875499722835)) ;
#49581=CARTESIAN_POINT('Ctrl Pts',(11.2454795765493,0.198027916508675,24.9806252339521)) ;
#49582=CARTESIAN_POINT('Ctrl Pts',(11.3019831172262,0.254531457185612,24.9674995088223)) ;
#49583=CARTESIAN_POINT('Ctrl Pts',(11.3377731498258,0.279106940985719,24.9604129001751)) ;
#49584=CARTESIAN_POINT('Ctrl Pts',(11.416519157157,0.311847989268857,24.9502865189927)) ;
#49585=CARTESIAN_POINT('Ctrl Pts',(11.459502635288,0.32,24.9474175425862)) ;
#49586=CARTESIAN_POINT('Ctrl Pts',(11.540497364712,0.32,24.9474175425862)) ;
#49587=CARTESIAN_POINT('Ctrl Pts',(11.583480842843,0.311847989268857,24.9502865189927)) ;
#49588=CARTESIAN_POINT('Ctrl Pts',(11.6622268501742,0.279106940985719,24.9604129001751)) ;
#49589=CARTESIAN_POINT('Ctrl Pts',(11.6980168827738,0.254531457185612,24.9674995088223)) ;
#49590=CARTESIAN_POINT('Ctrl Pts',(11.7545204234507,0.198027916508675,24.9806252339521)) ;
#49591=CARTESIAN_POINT('Ctrl Pts',(11.7791044225004,0.162233452253763,24.9875499722835)) ;
#49592=CARTESIAN_POINT('Ctrl Pts',(11.8118517942692,0.0834711465257763,
24.9972999591064)) ;
#49593=CARTESIAN_POINT('Ctrl Pts',(11.82,0.0404815515455362,25.)) ;
#49594=CARTESIAN_POINT('Ctrl Pts',(11.82,0.,25.)) ;
#49595=CARTESIAN_POINT('',(11.82,0.,23.)) ;
#49596=CARTESIAN_POINT('',(11.18,0.,23.)) ;
#49597=CARTESIAN_POINT('Ctrl Pts',(11.82,-6.93889390390723E-17,23.)) ;
#49598=CARTESIAN_POINT('Ctrl Pts',(11.82,0.0404815515455361,23.)) ;
#49599=CARTESIAN_POINT('Ctrl Pts',(11.8118517942692,0.0834711465257763,
23.0027000408936)) ;
#49600=CARTESIAN_POINT('Ctrl Pts',(11.7791044225004,0.162233452253763,23.0124500277165)) ;
#49601=CARTESIAN_POINT('Ctrl Pts',(11.7545204234507,0.198027916508675,23.0193747660479)) ;
#49602=CARTESIAN_POINT('Ctrl Pts',(11.6980168827738,0.254531457185612,23.0325004911777)) ;
#49603=CARTESIAN_POINT('Ctrl Pts',(11.6622268501742,0.279106940985719,23.0395870998249)) ;
#49604=CARTESIAN_POINT('Ctrl Pts',(11.583480842843,0.311847989268857,23.0497134810073)) ;
#49605=CARTESIAN_POINT('Ctrl Pts',(11.540497364712,0.32,23.0525824574138)) ;
#49606=CARTESIAN_POINT('Ctrl Pts',(11.459502635288,0.32,23.0525824574138)) ;
#49607=CARTESIAN_POINT('Ctrl Pts',(11.416519157157,0.311847989268857,23.0497134810073)) ;
#49608=CARTESIAN_POINT('Ctrl Pts',(11.3377731498258,0.279106940985719,23.0395870998249)) ;
#49609=CARTESIAN_POINT('Ctrl Pts',(11.3019831172262,0.254531457185612,23.0325004911777)) ;
#49610=CARTESIAN_POINT('Ctrl Pts',(11.2454795765493,0.198027916508675,23.0193747660479)) ;
#49611=CARTESIAN_POINT('Ctrl Pts',(11.2208955774996,0.162233452253763,23.0124500277165)) ;
#49612=CARTESIAN_POINT('Ctrl Pts',(11.1881482057308,0.0834711465257763,
23.0027000408936)) ;
#49613=CARTESIAN_POINT('Ctrl Pts',(11.18,0.0404815515455361,23.)) ;
#49614=CARTESIAN_POINT('Ctrl Pts',(11.18,0.,23.)) ;
#49615=CARTESIAN_POINT('Ctrl Pts',(11.18,1.80411241501588E-16,23.)) ;
#49616=CARTESIAN_POINT('Ctrl Pts',(11.18,-0.040481551545536,23.)) ;
#49617=CARTESIAN_POINT('Ctrl Pts',(11.1881482057308,-0.0834711465257763,
23.0027000408936)) ;
#49618=CARTESIAN_POINT('Ctrl Pts',(11.2208955774996,-0.162233452253763,
23.0124500277165)) ;
#49619=CARTESIAN_POINT('Ctrl Pts',(11.2454795765493,-0.198027916508675,
23.0193747660479)) ;
#49620=CARTESIAN_POINT('Ctrl Pts',(11.3019831172262,-0.254531457185612,
23.0325004911777)) ;
#49621=CARTESIAN_POINT('Ctrl Pts',(11.3377731498258,-0.279106940985719,
23.0395870998249)) ;
#49622=CARTESIAN_POINT('Ctrl Pts',(11.416519157157,-0.311847989268857,23.0497134810073)) ;
#49623=CARTESIAN_POINT('Ctrl Pts',(11.459502635288,-0.32,23.0525824574138)) ;
#49624=CARTESIAN_POINT('Ctrl Pts',(11.5,-0.32,23.0525824574138)) ;
#49625=CARTESIAN_POINT('Ctrl Pts',(11.540497364712,-0.32,23.0525824574138)) ;
#49626=CARTESIAN_POINT('Ctrl Pts',(11.583480842843,-0.311847989268857,23.0497134810073)) ;
#49627=CARTESIAN_POINT('Ctrl Pts',(11.6622268501742,-0.279106940985719,
23.0395870998249)) ;
#49628=CARTESIAN_POINT('Ctrl Pts',(11.6980168827738,-0.254531457185612,
23.0325004911777)) ;
#49629=CARTESIAN_POINT('Ctrl Pts',(11.7545204234507,-0.198027916508675,
23.0193747660479)) ;
#49630=CARTESIAN_POINT('Ctrl Pts',(11.7791044225004,-0.162233452253763,
23.0124500277165)) ;
#49631=CARTESIAN_POINT('Ctrl Pts',(11.8118517942692,-0.0834711465257763,
23.0027000408936)) ;
#49632=CARTESIAN_POINT('Ctrl Pts',(11.82,-0.0404815515455362,23.)) ;
#49633=CARTESIAN_POINT('Ctrl Pts',(11.82,-6.93889390390723E-18,23.)) ;
#49634=CARTESIAN_POINT('Origin',(4.5,0.,24.)) ;
#49635=CARTESIAN_POINT('Origin',(11.5,0.,24.)) ;
#49636=CARTESIAN_POINT('',(11.18,-3.91886975727153E-17,24.)) ;
#49637=CARTESIAN_POINT('Origin',(-11.5,0.,24.)) ;
#49638=CARTESIAN_POINT('',(-11.18,0.,23.)) ;
#49639=CARTESIAN_POINT('',(-11.82,0.,23.)) ;
#49640=CARTESIAN_POINT('Ctrl Pts',(-11.18,-6.24500451351651E-17,23.)) ;
#49641=CARTESIAN_POINT('Ctrl Pts',(-11.18,0.0404815515455361,23.)) ;
#49642=CARTESIAN_POINT('Ctrl Pts',(-11.1881482057308,0.0834711465257763,
23.0027000408936)) ;
#49643=CARTESIAN_POINT('Ctrl Pts',(-11.2208955774996,0.162233452253763,
23.0124500277165)) ;
#49644=CARTESIAN_POINT('Ctrl Pts',(-11.2454795765493,0.198027916508675,
23.0193747660479)) ;
#49645=CARTESIAN_POINT('Ctrl Pts',(-11.3019831172262,0.254531457185612,
23.0325004911777)) ;
#49646=CARTESIAN_POINT('Ctrl Pts',(-11.3377731498258,0.279106940985719,
23.0395870998249)) ;
#49647=CARTESIAN_POINT('Ctrl Pts',(-11.416519157157,0.311847989268857,23.0497134810073)) ;
#49648=CARTESIAN_POINT('Ctrl Pts',(-11.459502635288,0.32,23.0525824574138)) ;
#49649=CARTESIAN_POINT('Ctrl Pts',(-11.540497364712,0.32,23.0525824574138)) ;
#49650=CARTESIAN_POINT('Ctrl Pts',(-11.583480842843,0.311847989268857,23.0497134810073)) ;
#49651=CARTESIAN_POINT('Ctrl Pts',(-11.6622268501742,0.279106940985719,
23.0395870998249)) ;
#49652=CARTESIAN_POINT('Ctrl Pts',(-11.6980168827738,0.254531457185612,
23.0325004911777)) ;
#49653=CARTESIAN_POINT('Ctrl Pts',(-11.7545204234507,0.198027916508675,
23.0193747660479)) ;
#49654=CARTESIAN_POINT('Ctrl Pts',(-11.7791044225004,0.162233452253763,
23.0124500277165)) ;
#49655=CARTESIAN_POINT('Ctrl Pts',(-11.8118517942692,0.0834711465257763,
23.0027000408936)) ;
#49656=CARTESIAN_POINT('Ctrl Pts',(-11.82,0.0404815515455362,23.)) ;
#49657=CARTESIAN_POINT('Ctrl Pts',(-11.82,4.16333634234434E-17,23.)) ;
#49658=CARTESIAN_POINT('Ctrl Pts',(-11.82,2.08166817117217E-17,23.)) ;
#49659=CARTESIAN_POINT('Ctrl Pts',(-11.82,-0.0404815515455362,23.)) ;
#49660=CARTESIAN_POINT('Ctrl Pts',(-11.8118517942692,-0.0834711465257763,
23.0027000408936)) ;
#49661=CARTESIAN_POINT('Ctrl Pts',(-11.7791044225004,-0.162233452253763,
23.0124500277165)) ;
#49662=CARTESIAN_POINT('Ctrl Pts',(-11.7545204234507,-0.198027916508675,
23.0193747660479)) ;
#49663=CARTESIAN_POINT('Ctrl Pts',(-11.6980168827738,-0.254531457185612,
23.0325004911777)) ;
#49664=CARTESIAN_POINT('Ctrl Pts',(-11.6622268501742,-0.279106940985719,
23.0395870998249)) ;
#49665=CARTESIAN_POINT('Ctrl Pts',(-11.583480842843,-0.311847989268857,
23.0497134810073)) ;
#49666=CARTESIAN_POINT('Ctrl Pts',(-11.540497364712,-0.32,23.0525824574138)) ;
#49667=CARTESIAN_POINT('Ctrl Pts',(-11.5,-0.32,23.0525824574138)) ;
#49668=CARTESIAN_POINT('Ctrl Pts',(-11.459502635288,-0.32,23.0525824574138)) ;
#49669=CARTESIAN_POINT('Ctrl Pts',(-11.416519157157,-0.311847989268857,
23.0497134810073)) ;
#49670=CARTESIAN_POINT('Ctrl Pts',(-11.3377731498258,-0.279106940985719,
23.0395870998249)) ;
#49671=CARTESIAN_POINT('Ctrl Pts',(-11.3019831172262,-0.254531457185612,
23.0325004911777)) ;
#49672=CARTESIAN_POINT('Ctrl Pts',(-11.2454795765493,-0.198027916508675,
23.0193747660479)) ;
#49673=CARTESIAN_POINT('Ctrl Pts',(-11.2208955774996,-0.162233452253763,
23.0124500277165)) ;
#49674=CARTESIAN_POINT('Ctrl Pts',(-11.1881482057308,-0.0834711465257763,
23.0027000408936)) ;
#49675=CARTESIAN_POINT('Ctrl Pts',(-11.18,-0.040481551545536,23.)) ;
#49676=CARTESIAN_POINT('Ctrl Pts',(-11.18,1.80411241501588E-16,23.)) ;
#49677=CARTESIAN_POINT('',(-11.82,0.,25.)) ;
#49678=CARTESIAN_POINT('',(-11.82,-3.91886975727153E-17,24.)) ;
#49679=CARTESIAN_POINT('',(-11.18,0.,25.)) ;
#49680=CARTESIAN_POINT('Ctrl Pts',(-11.18,1.66533453693773E-16,25.)) ;
#49681=CARTESIAN_POINT('Ctrl Pts',(-11.18,-0.040481551545536,25.)) ;
#49682=CARTESIAN_POINT('Ctrl Pts',(-11.1881482057308,-0.0834711465257763,
24.9972999591064)) ;
#49683=CARTESIAN_POINT('Ctrl Pts',(-11.2208955774996,-0.162233452253763,
24.9875499722835)) ;
#49684=CARTESIAN_POINT('Ctrl Pts',(-11.2454795765493,-0.198027916508675,
24.9806252339521)) ;
#49685=CARTESIAN_POINT('Ctrl Pts',(-11.3019831172262,-0.254531457185612,
24.9674995088223)) ;
#49686=CARTESIAN_POINT('Ctrl Pts',(-11.3377731498258,-0.279106940985719,
24.9604129001751)) ;
#49687=CARTESIAN_POINT('Ctrl Pts',(-11.416519157157,-0.311847989268857,
24.9502865189927)) ;
#49688=CARTESIAN_POINT('Ctrl Pts',(-11.459502635288,-0.32,24.9474175425862)) ;
#49689=CARTESIAN_POINT('Ctrl Pts',(-11.5,-0.32,24.9474175425862)) ;
#49690=CARTESIAN_POINT('Ctrl Pts',(-11.540497364712,-0.32,24.9474175425862)) ;
#49691=CARTESIAN_POINT('Ctrl Pts',(-11.583480842843,-0.311847989268857,
24.9502865189927)) ;
#49692=CARTESIAN_POINT('Ctrl Pts',(-11.6622268501742,-0.279106940985719,
24.9604129001751)) ;
#49693=CARTESIAN_POINT('Ctrl Pts',(-11.6980168827738,-0.254531457185612,
24.9674995088223)) ;
#49694=CARTESIAN_POINT('Ctrl Pts',(-11.7545204234507,-0.198027916508675,
24.9806252339521)) ;
#49695=CARTESIAN_POINT('Ctrl Pts',(-11.7791044225004,-0.162233452253764,
24.9875499722835)) ;
#49696=CARTESIAN_POINT('Ctrl Pts',(-11.8118517942692,-0.0834711465257764,
24.9972999591064)) ;
#49697=CARTESIAN_POINT('Ctrl Pts',(-11.82,-0.0404815515455361,25.)) ;
#49698=CARTESIAN_POINT('Ctrl Pts',(-11.82,4.16333634234434E-17,25.)) ;
#49699=CARTESIAN_POINT('Ctrl Pts',(-11.82,-1.04083408558608E-17,25.)) ;
#49700=CARTESIAN_POINT('Ctrl Pts',(-11.82,0.0404815515455361,25.)) ;
#49701=CARTESIAN_POINT('Ctrl Pts',(-11.8118517942692,0.0834711465257764,
24.9972999591064)) ;
#49702=CARTESIAN_POINT('Ctrl Pts',(-11.7791044225004,0.162233452253763,
24.9875499722835)) ;
#49703=CARTESIAN_POINT('Ctrl Pts',(-11.7545204234507,0.198027916508675,
24.9806252339521)) ;
#49704=CARTESIAN_POINT('Ctrl Pts',(-11.6980168827738,0.254531457185612,
24.9674995088223)) ;
#49705=CARTESIAN_POINT('Ctrl Pts',(-11.6622268501742,0.279106940985719,
24.9604129001751)) ;
#49706=CARTESIAN_POINT('Ctrl Pts',(-11.583480842843,0.311847989268857,24.9502865189927)) ;
#49707=CARTESIAN_POINT('Ctrl Pts',(-11.540497364712,0.32,24.9474175425862)) ;
#49708=CARTESIAN_POINT('Ctrl Pts',(-11.459502635288,0.32,24.9474175425862)) ;
#49709=CARTESIAN_POINT('Ctrl Pts',(-11.416519157157,0.311847989268857,24.9502865189927)) ;
#49710=CARTESIAN_POINT('Ctrl Pts',(-11.3377731498258,0.279106940985719,
24.9604129001751)) ;
#49711=CARTESIAN_POINT('Ctrl Pts',(-11.3019831172262,0.254531457185612,
24.9674995088223)) ;
#49712=CARTESIAN_POINT('Ctrl Pts',(-11.2454795765493,0.198027916508675,
24.9806252339521)) ;
#49713=CARTESIAN_POINT('Ctrl Pts',(-11.2208955774996,0.162233452253763,
24.9875499722835)) ;
#49714=CARTESIAN_POINT('Ctrl Pts',(-11.1881482057308,0.0834711465257763,
24.9972999591064)) ;
#49715=CARTESIAN_POINT('Ctrl Pts',(-11.18,0.040481551545536,25.)) ;
#49716=CARTESIAN_POINT('Ctrl Pts',(-11.18,-1.66533453693773E-16,25.)) ;
#49717=CARTESIAN_POINT('Origin',(-4.5,0.,24.)) ;
#49718=CARTESIAN_POINT('',(-4.5,0.,23.)) ;
#49719=CARTESIAN_POINT('',(-4.5,0.,25.)) ;
#49720=CARTESIAN_POINT('',(-4.5,0.,24.)) ;
#49721=CARTESIAN_POINT('Origin',(-4.5,0.,24.)) ;
#49722=CARTESIAN_POINT('Origin',(-8.25,0.,24.)) ;
#49723=CARTESIAN_POINT('Origin',(-4.5,0.,24.)) ;
#49724=CARTESIAN_POINT('',(-8.25,-1.22464679914735E-16,25.)) ;
#49725=CARTESIAN_POINT('',(-12.,-1.22464679914735E-16,25.)) ;
#49726=CARTESIAN_POINT('',(-8.25,-1.22464679914735E-16,25.)) ;
#49727=CARTESIAN_POINT('Origin',(-12.,0.,24.)) ;
#49728=CARTESIAN_POINT('Origin',(-12.,0.,24.)) ;
#49729=CARTESIAN_POINT('Origin',(-4.5,0.,24.)) ;
#49730=CARTESIAN_POINT('Origin',(0.,0.,24.)) ;
#49731=CARTESIAN_POINT('',(0.,-4.5,24.8)) ;
#49732=CARTESIAN_POINT('',(2.75545529808154E-16,-4.5,25.5)) ;
#49733=CARTESIAN_POINT('',(2.75545529808154E-16,-4.5,24.)) ;
#49734=CARTESIAN_POINT('',(0.,-4.5,23.2)) ;
#49735=CARTESIAN_POINT('',(0.,-4.5,24.)) ;
#49736=CARTESIAN_POINT('',(2.75545529808154E-16,-4.5,22.5)) ;
#49737=CARTESIAN_POINT('',(2.75545529808154E-16,-4.5,24.)) ;
#49738=CARTESIAN_POINT('',(-4.5,-5.51091059616309E-16,22.5)) ;
#49739=CARTESIAN_POINT('Origin',(0.,0.,22.5)) ;
#49740=CARTESIAN_POINT('',(-4.5,0.,23.)) ;
#49741=CARTESIAN_POINT('',(-4.5,-5.51091059616309E-16,24.)) ;
#49742=CARTESIAN_POINT('',(-4.5,0.,25.)) ;
#49743=CARTESIAN_POINT('',(-4.5,0.,24.)) ;
#49744=CARTESIAN_POINT('',(-4.5,-5.51091059616309E-16,25.5)) ;
#49745=CARTESIAN_POINT('',(-4.5,-5.51091059616309E-16,24.)) ;
#49746=CARTESIAN_POINT('Origin',(0.,0.,25.5)) ;
#49747=CARTESIAN_POINT('',(4.5,0.,23.)) ;
#49748=CARTESIAN_POINT('',(4.5,0.,25.)) ;
#49749=CARTESIAN_POINT('',(4.5,0.,24.)) ;
#49750=CARTESIAN_POINT('Origin',(0.,0.,25.5)) ;
#49751=CARTESIAN_POINT('Origin',(0.,0.,25.5)) ;
#49752=CARTESIAN_POINT('',(-3.5,4.28626379701574E-16,25.5)) ;
#49753=CARTESIAN_POINT('Origin',(0.,0.,25.5)) ;
#49754=CARTESIAN_POINT('Origin',(0.,0.,22.5)) ;
#49755=CARTESIAN_POINT('Origin',(0.,0.,22.5)) ;
#49756=CARTESIAN_POINT('',(-3.5,-4.28626379701574E-16,22.5)) ;
#49757=CARTESIAN_POINT('Origin',(0.,0.,22.5)) ;
#49758=CARTESIAN_POINT('Origin',(0.,0.,24.)) ;
#49759=CARTESIAN_POINT('Origin',(0.,0.,24.)) ;
#49760=CARTESIAN_POINT('',(-3.5,-4.28626379701574E-16,24.)) ;
#50375=UNCERTAINTY_MEASURE_WITH_UNIT(LENGTH_MEASURE(0.001),#50441,
'DISTANCE_ACCURACY_VALUE',
'Maximum model space distance between geometric entities at asserted c
onnectivities') ;
#50387=UNCERTAINTY_MEASURE_WITH_UNIT(LENGTH_MEASURE(0.001),#50441,
'DISTANCE_ACCURACY_VALUE',
'Maximum model space distance between geometric entities at asserted c
onnectivities') ;
#50428=(
GEOMETRIC_REPRESENTATION_CONTEXT(3)
GLOBAL_UNCERTAINTY_ASSIGNED_CONTEXT((#50375))
GLOBAL_UNIT_ASSIGNED_CONTEXT((#50441,#50443,#50444))
REPRESENTATION_CONTEXT('','3D')
) ;
#50440=(
GEOMETRIC_REPRESENTATION_CONTEXT(3)
GLOBAL_UNCERTAINTY_ASSIGNED_CONTEXT((#50387))
GLOBAL_UNIT_ASSIGNED_CONTEXT((#50441,#50443,#50444))
REPRESENTATION_CONTEXT('','3D')
) ;
#50441=(
LENGTH_UNIT()
NAMED_UNIT(*)
SI_UNIT(.CENTI.,.METRE.)
) ;
#50443=(
NAMED_UNIT(*)
PLANE_ANGLE_UNIT()
SI_UNIT($,.RADIAN.)
) ;
#50444=(
NAMED_UNIT(*)
SI_UNIT($,.STERADIAN.)
SOLID_ANGLE_UNIT()
) ;
#50485=SHAPE_DEFINITION_REPRESENTATION(#50575,#50659) ;
#50575=PRODUCT_DEFINITION_SHAPE('',$,#50712) ;
#50659=SHAPE_REPRESENTATION('',(#32118),#50428) ;
#50671=PRODUCT_DEFINITION_CONTEXT('part definition',#50829,'design') ;
#50712=PRODUCT_DEFINITION('PENDULUM_TRUNNION_YOKE',
'PENDULUM_TRUNNION_YOKE',#50764,#50671) ;
#50764=PRODUCT_DEFINITION_FORMATION('',$,#50871) ;
#50829=APPLICATION_CONTEXT(
'Core Data for Automotive Mechanical Design Process') ;
#50830=PRODUCT_CONTEXT('part definition',#50829,'mechanical') ;
#50871=PRODUCT('PENDULUM_TRUNNION_YOKE','PENDULUM_TRUNNION_YOKE',$,(#50830)) ;
#50883=PRESENTATION_STYLE_ASSIGNMENT((#50890)) ;
#50890=SURFACE_STYLE_USAGE(.BOTH.,#50897) ;
#50897=SURFACE_SIDE_STYLE('',(#50904)) ;
#50904=SURFACE_STYLE_FILL_AREA(#50911) ;
#50911=FILL_AREA_STYLE('Steel - Satin',(#50918)) ;
#50918=FILL_AREA_STYLE_COLOUR('Steel - Satin',#50925) ;
#50925=COLOUR_RGB('Steel - Satin', 0.31764706, 0.68627451, 0.89019608) ;
ENDSEC;
END-ISO-10303-21;
